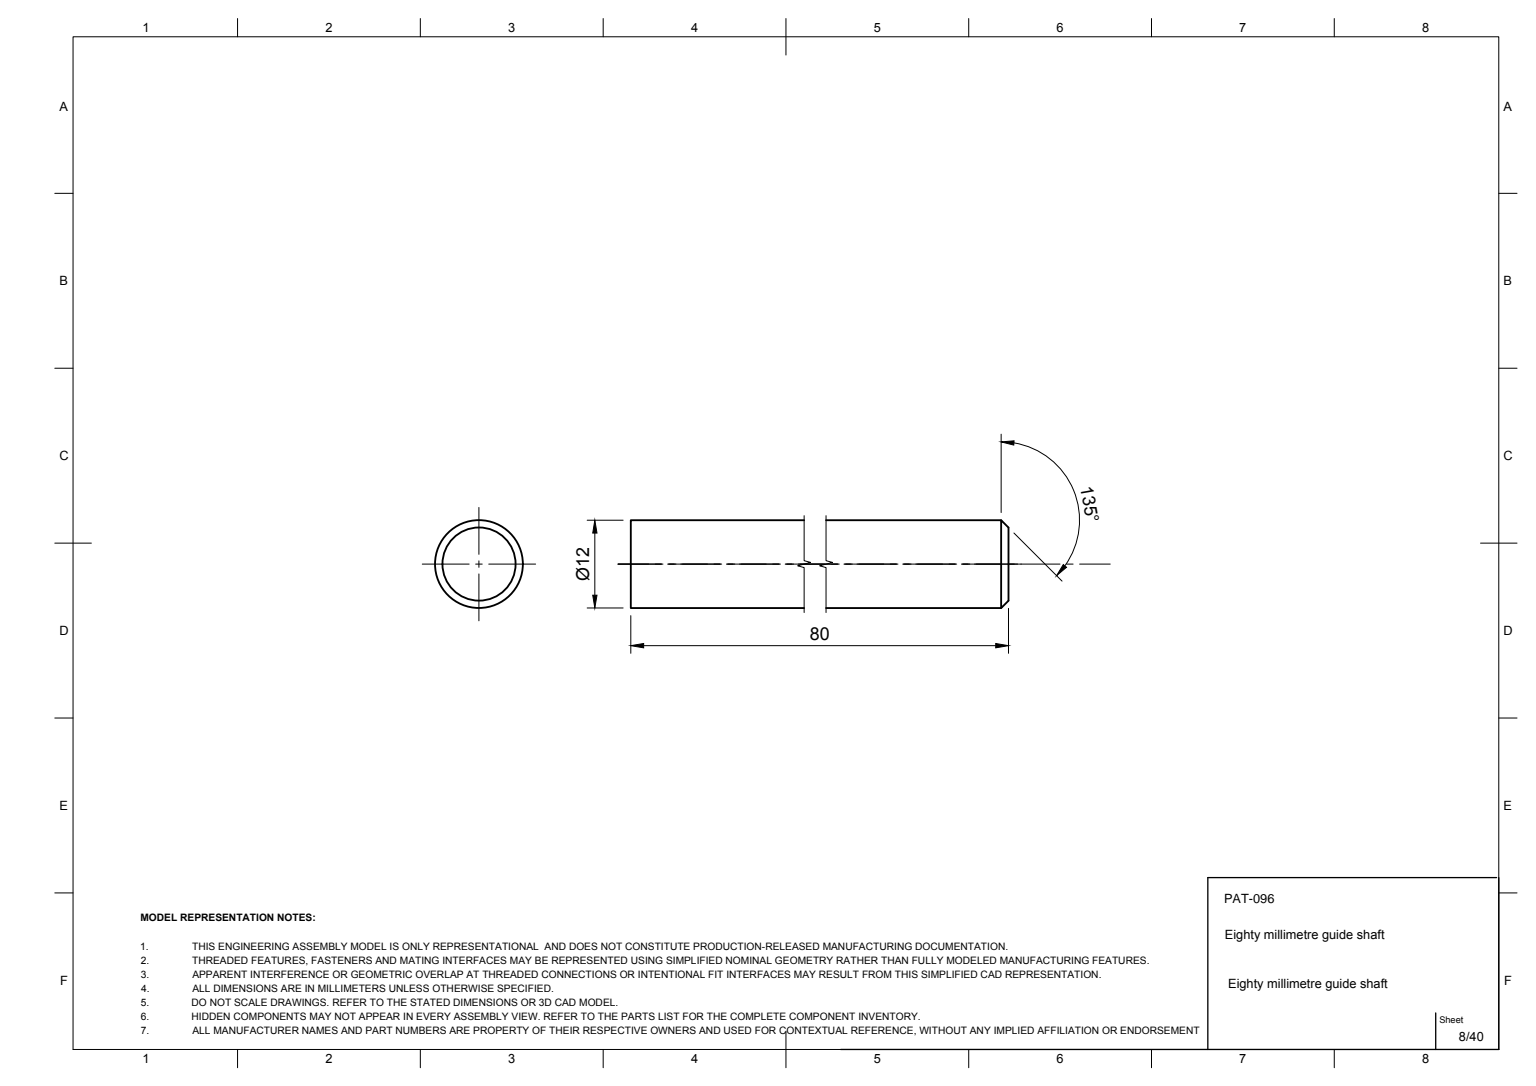
ISO-10303-21;
HEADER;
/* Generated by software containing ST-Developer
 * from STEP Tools, Inc. (www.steptools.com) 
 */

FILE_DESCRIPTION(
/* description */ ('PAT-096'),
/* implementation_level */ '2;1');

FILE_NAME(
/* name */ 'Eighty millimetre guide shaft.step',
/* time_stamp */ '2026-10-29T17:03:14-07:00',
/* author */ (''),
/* organization */ (''),
/* preprocessor_version */ 'ST-DEVELOPER v20.2',
/* originating_system */ 'Autodesk Translation Framework v15.17.0.0',
/* authorisation */ '');

FILE_SCHEMA (('AUTOMOTIVE_DESIGN { 1 0 10303 214 3 1 1 }'));
ENDSEC;

DATA;
#10=MECHANICAL_DESIGN_GEOMETRIC_PRESENTATION_REPRESENTATION('',(#415),#10650);
#319=CONICAL_SURFACE('',#6220,0.55,0.785398163397448);
#345=SHAPE_REPRESENTATION_RELATIONSHIP('SRR','None',#10806,#376);
#376=ADVANCED_BREP_SHAPE_REPRESENTATION('',(#453),#10624);
#415=STYLED_ITEM('',(#11064),#453);
#453=MANIFOLD_SOLID_BREP('Body1',#5549);
#665=PLANE('',#6218);
#666=PLANE('',#6224);
#918=FACE_OUTER_BOUND('',#1313,.T.);
#919=FACE_OUTER_BOUND('',#1314,.T.);
#920=FACE_OUTER_BOUND('',#1315,.T.);
#921=FACE_OUTER_BOUND('',#1316,.T.);
#1313=EDGE_LOOP('',(#4255));
#1314=EDGE_LOOP('',(#4256,#4257,#4258,#4259));
#1315=EDGE_LOOP('',(#4260,#4261,#4262,#4263));
#1316=EDGE_LOOP('',(#4264));
#1692=LINE('',#9530,#2021);
#1693=LINE('',#9533,#2022);
#2021=VECTOR('',#7376,0.55);
#2022=VECTOR('',#7381,0.6);
#2416=CIRCLE('',#6219,0.6);
#2417=CIRCLE('',#6221,0.6);
#2418=CIRCLE('',#6222,0.5);
#2767=VERTEX_POINT('',#9524);
#2768=VERTEX_POINT('',#9527);
#2769=VERTEX_POINT('',#9529);
#3306=EDGE_CURVE('',#2767,#2767,#2416,.T.);
#3307=EDGE_CURVE('',#2768,#2768,#2417,.T.);
#3308=EDGE_CURVE('',#2768,#2769,#1692,.T.);
#3309=EDGE_CURVE('',#2769,#2769,#2418,.T.);
#3310=EDGE_CURVE('',#2767,#2768,#1693,.T.);
#4255=ORIENTED_EDGE('',*,*,#3306,.F.);
#4256=ORIENTED_EDGE('',*,*,#3307,.T.);
#4257=ORIENTED_EDGE('',*,*,#3308,.T.);
#4258=ORIENTED_EDGE('',*,*,#3309,.T.);
#4259=ORIENTED_EDGE('',*,*,#3308,.F.);
#4260=ORIENTED_EDGE('',*,*,#3306,.T.);
#4261=ORIENTED_EDGE('',*,*,#3310,.T.);
#4262=ORIENTED_EDGE('',*,*,#3307,.F.);
#4263=ORIENTED_EDGE('',*,*,#3310,.F.);
#4264=ORIENTED_EDGE('',*,*,#3309,.F.);
#5123=CYLINDRICAL_SURFACE('',#6223,0.6);
#5323=ADVANCED_FACE('',(#918),#665,.T.);
#5324=ADVANCED_FACE('',(#919),#319,.T.);
#5325=ADVANCED_FACE('',(#920),#5123,.T.);
#5326=ADVANCED_FACE('',(#921),#666,.F.);
#5549=CLOSED_SHELL('',(#5323,#5324,#5325,#5326));
#6217=AXIS2_PLACEMENT_3D('',#9522,#7366,#7367);
#6218=AXIS2_PLACEMENT_3D('',#9523,#7368,#7369);
#6219=AXIS2_PLACEMENT_3D('',#9525,#7370,#7371);
#6220=AXIS2_PLACEMENT_3D('',#9526,#7372,#7373);
#6221=AXIS2_PLACEMENT_3D('',#9528,#7374,#7375);
#6222=AXIS2_PLACEMENT_3D('',#9531,#7377,#7378);
#6223=AXIS2_PLACEMENT_3D('',#9532,#7379,#7380);
#6224=AXIS2_PLACEMENT_3D('',#9534,#7382,#7383);
#7366=DIRECTION('axis',(0.,0.,1.));
#7367=DIRECTION('refdir',(1.,0.,0.));
#7368=DIRECTION('center_axis',(1.,0.,0.));
#7369=DIRECTION('ref_axis',(0.,0.,-1.));
#7370=DIRECTION('center_axis',(-1.,0.,0.));
#7371=DIRECTION('ref_axis',(0.,0.,-1.));
#7372=DIRECTION('center_axis',(1.,0.,0.));
#7373=DIRECTION('ref_axis',(0.,0.,-1.));
#7374=DIRECTION('center_axis',(-1.,0.,0.));
#7375=DIRECTION('ref_axis',(0.,0.,-1.));
#7376=DIRECTION('',(-0.707106781186548,8.65956056235493E-17,-0.707106781186547));
#7377=DIRECTION('center_axis',(1.,0.,0.));
#7378=DIRECTION('ref_axis',(0.,0.,-1.));
#7379=DIRECTION('center_axis',(1.,0.,0.));
#7380=DIRECTION('ref_axis',(0.,0.,-1.));
#7381=DIRECTION('',(-1.,0.,0.));
#7382=DIRECTION('center_axis',(1.,0.,0.));
#7383=DIRECTION('ref_axis',(0.,0.,-1.));
#9522=CARTESIAN_POINT('',(0.,0.,0.));
#9523=CARTESIAN_POINT('Origin',(8.,0.,0.));
#9524=CARTESIAN_POINT('',(8.,7.34788079488412E-17,0.6));
#9525=CARTESIAN_POINT('Origin',(8.,0.,0.));
#9526=CARTESIAN_POINT('Origin',(0.05,0.,0.));
#9527=CARTESIAN_POINT('',(0.1,7.34788079488412E-17,0.6));
#9528=CARTESIAN_POINT('Origin',(0.1,0.,0.));
#9529=CARTESIAN_POINT('',(0.,-6.12323399573677E-17,0.5));
#9530=CARTESIAN_POINT('',(0.05,-6.73555739531044E-17,0.55));
#9531=CARTESIAN_POINT('Origin',(0.,0.,0.));
#9532=CARTESIAN_POINT('Origin',(0.,0.,0.));
#9533=CARTESIAN_POINT('',(0.,-7.34788079488412E-17,0.6));
#9534=CARTESIAN_POINT('Origin',(0.,0.,0.));
#10585=UNCERTAINTY_MEASURE_WITH_UNIT(LENGTH_MEASURE(0.001),#10651,
'DISTANCE_ACCURACY_VALUE',
'Maximum model space distance between geometric entities at asserted c
onnectivities');
#10611=UNCERTAINTY_MEASURE_WITH_UNIT(LENGTH_MEASURE(0.001),#10651,
'DISTANCE_ACCURACY_VALUE',
'Maximum model space distance between geometric entities at asserted c
onnectivities');
#10624=(
GEOMETRIC_REPRESENTATION_CONTEXT(3)
GLOBAL_UNCERTAINTY_ASSIGNED_CONTEXT((#10585))
GLOBAL_UNIT_ASSIGNED_CONTEXT((#10651,#10653,#10654))
REPRESENTATION_CONTEXT('','3D')
);
#10650=(
GEOMETRIC_REPRESENTATION_CONTEXT(3)
GLOBAL_UNCERTAINTY_ASSIGNED_CONTEXT((#10611))
GLOBAL_UNIT_ASSIGNED_CONTEXT((#10651,#10653,#10654))
REPRESENTATION_CONTEXT('','3D')
);
#10651=(
LENGTH_UNIT()
NAMED_UNIT(*)
SI_UNIT(.CENTI.,.METRE.)
);
#10653=(
NAMED_UNIT(*)
PLANE_ANGLE_UNIT()
SI_UNIT($,.RADIAN.)
);
#10654=(
NAMED_UNIT(*)
SI_UNIT($,.STERADIAN.)
SOLID_ANGLE_UNIT()
);
#10667=SHAPE_DEFINITION_REPRESENTATION(#10710,#10806);
#10710=PRODUCT_DEFINITION_SHAPE('',$,#10845);
#10806=SHAPE_REPRESENTATION('',(#6217),#10624);
#10832=PRODUCT_DEFINITION_CONTEXT('part definition',#10948,'design');
#10845=PRODUCT_DEFINITION('Eighty millimetre guide shaft',
'Eighty millimetre guide shaft',#10883,#10832);
#10883=PRODUCT_DEFINITION_FORMATION('',$,#10962);
#10948=APPLICATION_CONTEXT(
'Core Data for Automotive Mechanical Design Process');
#10949=PRODUCT_CONTEXT('part definition',#10948,'mechanical');
#10962=PRODUCT('Eighty millimetre guide shaft',
'Eighty millimetre guide shaft','Eighty millimetre guide shaft',(#10949));
#11058=COLOUR_RGB('Grey',0.48,0.52,0.57);
#11059=FILL_AREA_STYLE_COLOUR('',#11058);
#11060=FILL_AREA_STYLE('',(#11059));
#11061=SURFACE_STYLE_FILL_AREA(#11060);
#11062=SURFACE_SIDE_STYLE('',(#11061));
#11063=SURFACE_STYLE_USAGE(.BOTH.,#11062);
#11064=PRESENTATION_STYLE_ASSIGNMENT((#11063));
ENDSEC;
END-ISO-10303-21;
